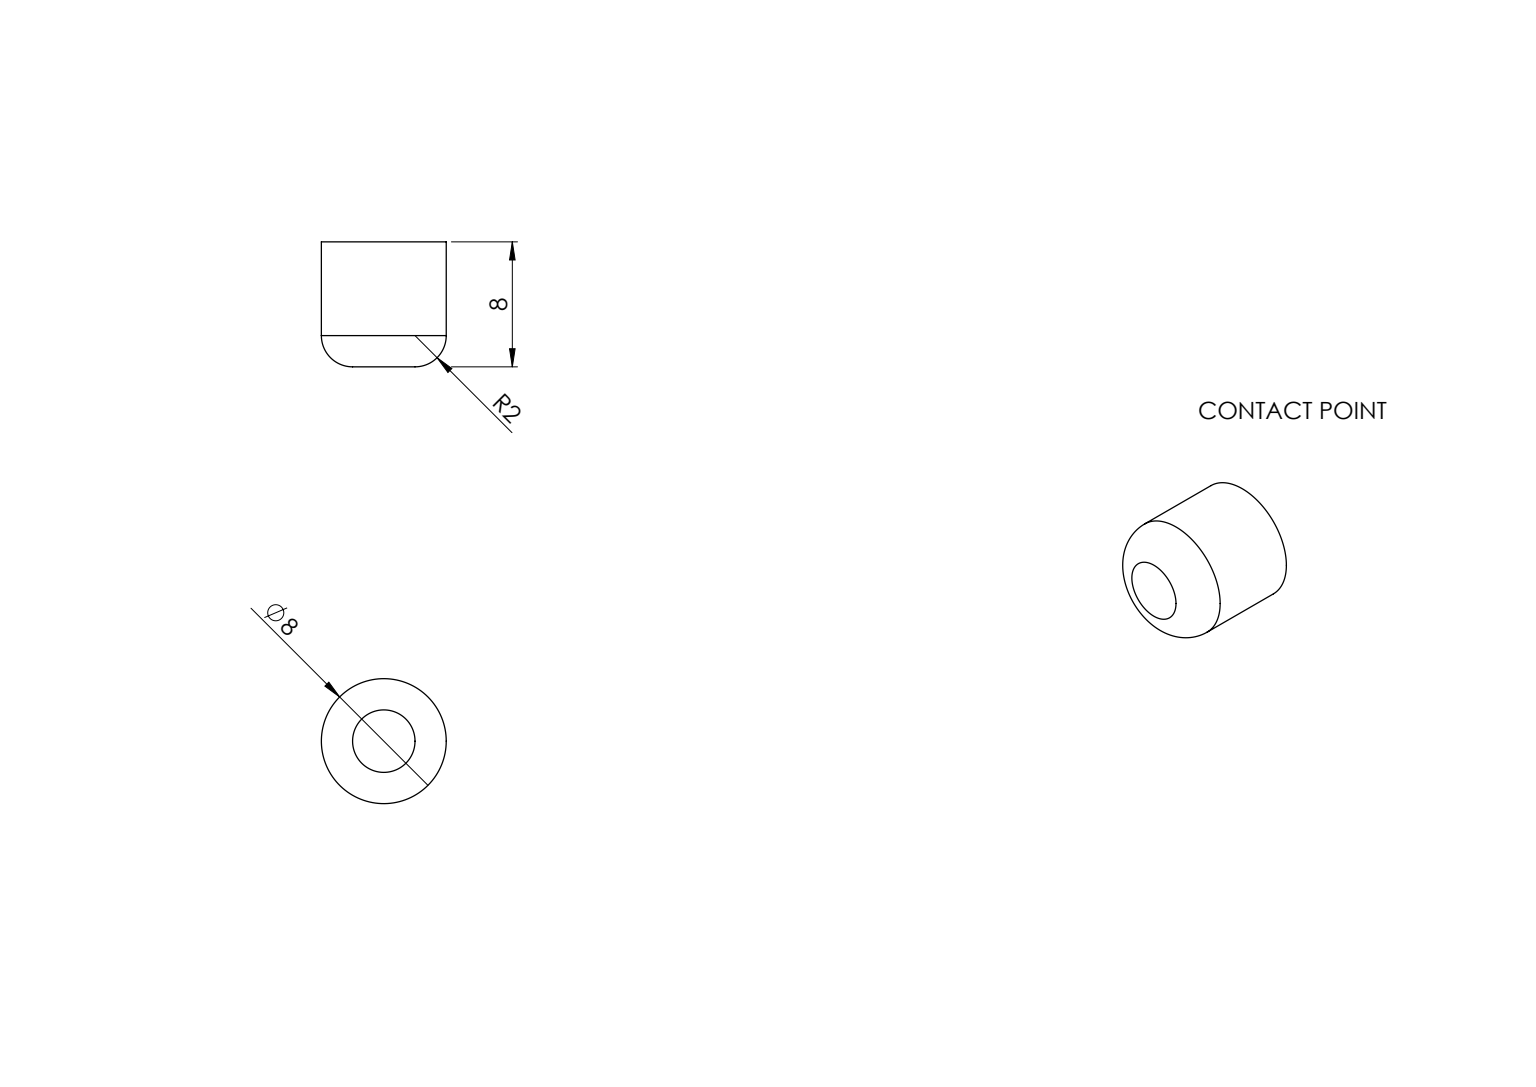
ISO-10303-21;
HEADER;
FILE_DESCRIPTION (('STEP AP214'),
    '1' );
FILE_NAME ('contact point.step',
    '2026-10-26T12:50:16',
    ( '' ),
    ( '' ),
    'SwSTEP 2.0',
    'SolidWorks 2026',
    '' );
FILE_SCHEMA (( 'AUTOMOTIVE_DESIGN' ));
ENDSEC;

DATA;
#29=ORIENTED_EDGE ( 'NONE', *, *, #15667, .T. ) ;
#56=VERTEX_POINT ( 'NONE', #24269 ) ;
#75=TOROIDAL_SURFACE ( 'NONE', #19699, 2.000000000000000000, 2.000000000000000000 ) ;
#102=ADVANCED_FACE ( 'NONE', ( #22181 ), #12564, .T. ) ;
#110=CARTESIAN_POINT ( 'NONE',  ( 1.500000000000001776, -10.49999999999999289, 4.999999999999993783 ) ) ;
#186=ORIENTED_EDGE ( 'NONE', *, *, #6669, .T. ) ;
#197=EDGE_CURVE ( 'NONE', #20602, #23121, #20077, .T. ) ;
#412=ORIENTED_EDGE ( 'NONE', *, *, #15667, .F. ) ;
#459=( GEOMETRIC_REPRESENTATION_CONTEXT ( 3 ) GLOBAL_UNCERTAINTY_ASSIGNED_CONTEXT ( ( #10970 ) ) GLOBAL_UNIT_ASSIGNED_CONTEXT ( ( #23012, #3129, #18575 ) ) REPRESENTATION_CONTEXT ( 'NONE', 'WORKASPACE' ) );
#546=EDGE_CURVE ( 'NONE', #10805, #16184, #12212, .T. ) ;
#620=EDGE_CURVE ( 'NONE', #5209, #6382, #2280, .T. ) ;
#698=ORIENTED_EDGE ( 'NONE', *, *, #8966, .F. ) ;
#734=LINE ( 'NONE', #6878, #984 ) ;
#738=FILL_AREA_STYLE_COLOUR ( '', #17309 ) ;
#806=AXIS2_PLACEMENT_3D ( 'NONE', #20605, #12487, #857 ) ;
#857=DIRECTION ( 'NONE',  ( -1.000000000000000000, 0.000000000000000000, 0.000000000000000000 ) ) ;
#871=SHAPE_REPRESENTATION_RELATIONSHIP ( 'NONE' , 'NONE' ,  #23343, #13495 ) ;
#935=ORIENTED_EDGE ( 'NONE', *, *, #9732, .T. ) ;
#984=VECTOR ( 'NONE', #20472, 1000.000000000000000 ) ;
#1087=VERTEX_POINT ( 'NONE', #6518 ) ;
#1292=UNCERTAINTY_MEASURE_WITH_UNIT (LENGTH_MEASURE( 1.000000000000000082E-05 ), #12896, 'distance_accuracy_value', 'NONE');
#1392=PRODUCT_CONTEXT ( 'NONE', #10427, 'mechanical' ) ;
#1414=ORIENTED_EDGE ( 'NONE', *, *, #7433, .F. ) ;
#1426=MECHANICAL_DESIGN_GEOMETRIC_PRESENTATION_REPRESENTATION('',(#12709),#8113);
#1448=EDGE_LOOP ( 'NONE', ( #25041, #5384, #21791, #23680 ) ) ;
#1535=ORIENTED_EDGE ( 'NONE', *, *, #10759, .F. ) ;
#1546=DIRECTION ( 'NONE',  ( 1.000000000000000000, 0.000000000000000000, 0.000000000000000000 ) ) ;
#1618=EDGE_LOOP ( 'NONE', ( #2456, #10455, #25171, #2324 ) ) ;
#2076=DIRECTION ( 'NONE',  ( 0.000000000000000000, -1.000000000000000000, 0.000000000000000000 ) ) ;
#2122=EDGE_CURVE ( 'NONE', #23121, #13852, #15327, .T. ) ;
#2130=CARTESIAN_POINT ( 'NONE',  ( 4.000000000000003553, -8.999999999999992895, 0.000000000000000000 ) ) ;
#2280=LINE ( 'NONE', #19913, #10677 ) ;
#2308=DIRECTION ( 'NONE',  ( 1.000000000000000000, 0.000000000000000000, 0.000000000000000000 ) ) ;
#2324=ORIENTED_EDGE ( 'NONE', *, *, #620, .F. ) ;
#2456=ORIENTED_EDGE ( 'NONE', *, *, #23666, .F. ) ;
#2478=CARTESIAN_POINT ( 'NONE',  ( 1.500000000000001776, -7.499999999999993783, -6.938893903907228378E-15 ) ) ;
#2560=VECTOR ( 'NONE', #24669, 1000.000000000000000 ) ;
#2573=( NAMED_UNIT ( * ) SI_UNIT ( $, .STERADIAN. ) SOLID_ANGLE_UNIT ( ) );
#2605=EDGE_LOOP ( 'NONE', ( #20644, #21893 ) ) ;
#2676=( GEOMETRIC_REPRESENTATION_CONTEXT ( 3 ) GLOBAL_UNCERTAINTY_ASSIGNED_CONTEXT ( ( #12808 ) ) GLOBAL_UNIT_ASSIGNED_CONTEXT ( ( #3892, #25726, #22442 ) ) REPRESENTATION_CONTEXT ( 'NONE', 'WORKASPACE' ) );
#2786=CARTESIAN_POINT ( 'NONE',  ( 3.469446951953614189E-15, -8.999999999999992895, 6.000000000000000000 ) ) ;
#2807=CARTESIAN_POINT ( 'NONE',  ( 3.469446951953614189E-15, -8.999999999999992895, 0.000000000000000000 ) ) ;
#2920=ORIENTED_EDGE ( 'NONE', *, *, #2122, .F. ) ;
#2933=CIRCLE ( 'NONE', #15893, 4.000000000000000000 ) ;
#2940=EDGE_CURVE ( 'NONE', #20602, #3531, #10020, .T. ) ;
#2999=AXIS2_PLACEMENT_3D ( 'NONE', #9884, #3615, #11585 ) ;
#3099=ADVANCED_FACE ( 'NONE', ( #25038, #19143 ), #9217, .F. ) ;
#3100=DIRECTION ( 'NONE',  ( 0.000000000000000000, 0.000000000000000000, 1.000000000000000000 ) ) ;
#3129=( NAMED_UNIT ( * ) PLANE_ANGLE_UNIT ( ) SI_UNIT ( $, .RADIAN. ) );
#3313=EDGE_LOOP ( 'NONE', ( #412, #21152, #3951, #4447 ) ) ;
#3349=CARTESIAN_POINT ( 'NONE',  ( 1.500000000000001776, -7.499999999999993783, 4.999999999999993783 ) ) ;
#3531=VERTEX_POINT ( 'NONE', #23628 ) ;
#3615=DIRECTION ( 'NONE',  ( -0.000000000000000000, -0.000000000000000000, -1.000000000000000000 ) ) ;
#3722=PRODUCT_DEFINITION ( 'UNKNOWN', '', #21072, #20916 ) ;
#3755=DIRECTION ( 'NONE',  ( 0.000000000000000000, 1.000000000000000000, 0.000000000000000000 ) ) ;
#3773=EDGE_LOOP ( 'NONE', ( #1414, #13122, #6814, #9882 ) ) ;
#3789=LINE ( 'NONE', #9159, #13919 ) ;
#3892=( LENGTH_UNIT ( ) NAMED_UNIT ( * ) SI_UNIT ( .MILLI., .METRE. ) );
#3951=ORIENTED_EDGE ( 'NONE', *, *, #2122, .T. ) ;
#4029=PLANE ( 'NONE',  #25126 ) ;
#4157=DIRECTION ( 'NONE',  ( -1.000000000000000000, 0.000000000000000000, 0.000000000000000000 ) ) ;
#4231=CIRCLE ( 'NONE', #6325, 2.000000000000000000 ) ;
#4279=LINE ( 'NONE', #110, #15026 ) ;
#4314=DIRECTION ( 'NONE',  ( 1.000000000000000000, -0.000000000000000000, -0.000000000000000000 ) ) ;
#4383=EDGE_LOOP ( 'NONE', ( #19500, #13715, #698, #5012 ) ) ;
#4403=CYLINDRICAL_SURFACE ( 'NONE', #8424, 4.000000000000000000 ) ;
#4447=ORIENTED_EDGE ( 'NONE', *, *, #10150, .T. ) ;
#4601=DIRECTION ( 'NONE',  ( 0.000000000000000000, 1.000000000000000000, 0.000000000000000000 ) ) ;
#4751=CARTESIAN_POINT ( 'NONE',  ( 1.500000000000001776, -10.49999999999999289, -6.938893903907228378E-15 ) ) ;
#4765=FACE_OUTER_BOUND ( 'NONE', #4383, .T. ) ;
#4835=FACE_OUTER_BOUND ( 'NONE', #1448, .T. ) ;
#4917=FACE_OUTER_BOUND ( 'NONE', #9792, .T. ) ;
#5012=ORIENTED_EDGE ( 'NONE', *, *, #2940, .F. ) ;
#5149=DIRECTION ( 'NONE',  ( 0.000000000000000000, 0.000000000000000000, 1.000000000000000000 ) ) ;
#5173=DIRECTION ( 'NONE',  ( 0.000000000000000000, 0.000000000000000000, 1.000000000000000000 ) ) ;
#5209=VERTEX_POINT ( 'NONE', #6579 ) ;
#5233=EDGE_CURVE ( 'NONE', #5209, #1087, #7239, .T. ) ;
#5384=ORIENTED_EDGE ( 'NONE', *, *, #5233, .F. ) ;
#5442=MECHANICAL_DESIGN_GEOMETRIC_PRESENTATION_REPRESENTATION('',(#23407),#459);
#5468=DIRECTION ( 'NONE',  ( 0.000000000000000000, 0.000000000000000000, 1.000000000000000000 ) ) ;
#5632=DIRECTION ( 'NONE',  ( 0.000000000000000000, 0.000000000000000000, 1.000000000000000000 ) ) ;
#5687=EDGE_CURVE ( 'NONE', #7768, #17145, #734, .T. ) ;
#5822=FACE_OUTER_BOUND ( 'NONE', #12954, .T. ) ;
#5941=CARTESIAN_POINT ( 'NONE',  ( 1.500000000000001776, -7.499999999999993783, 4.999999999999993783 ) ) ;
#5971=DIRECTION ( 'NONE',  ( -0.000000000000000000, -0.000000000000000000, -1.000000000000000000 ) ) ;
#5983=PLANE ( 'NONE',  #22192 ) ;
#6120=CARTESIAN_POINT ( 'NONE',  ( 1.500000000000001776, -10.49999999999999289, 4.999999999999993783 ) ) ;
#6325=AXIS2_PLACEMENT_3D ( 'NONE', #13043, #3100, #11959 ) ;
#6372=CARTESIAN_POINT ( 'NONE',  ( 3.469446951953614189E-15, -8.999999999999992895, 8.000000000000000000 ) ) ;
#6382=VERTEX_POINT ( 'NONE', #15341 ) ;
#6402=CARTESIAN_POINT ( 'NONE',  ( -3.999999999999996447, -8.999999999999992895, 6.000000000000000000 ) ) ;
#6518=CARTESIAN_POINT ( 'NONE',  ( -1.499999999999998224, -10.49999999999999289, -6.938893903907228378E-15 ) ) ;
#6579=CARTESIAN_POINT ( 'NONE',  ( -1.499999999999998224, -10.49999999999999289, 4.999999999999993783 ) ) ;
#6629=CARTESIAN_POINT ( 'NONE',  ( 3.469446951953614189E-15, -8.999999999999992895, 8.000000000000000000 ) ) ;
#6669=EDGE_CURVE ( 'NONE', #23121, #20602, #23055, .T. ) ;
#6814=ORIENTED_EDGE ( 'NONE', *, *, #12872, .T. ) ;
#6878=CARTESIAN_POINT ( 'NONE',  ( 1.500000000000001776, -7.499999999999993783, -6.938893903907228378E-15 ) ) ;
#6882=SURFACE_STYLE_USAGE ( .BOTH. , #8708 ) ;
#6884=CARTESIAN_POINT ( 'NONE',  ( -1.499999999999998224, -10.49999999999999289, 4.999999999999993783 ) ) ;
#6906=ADVANCED_FACE ( 'NONE', ( #4765 ), #75, .T. ) ;
#7004=( NAMED_UNIT ( * ) PLANE_ANGLE_UNIT ( ) SI_UNIT ( $, .RADIAN. ) );
#7052=AXIS2_PLACEMENT_3D ( 'NONE', #21524, #21788, #15381 ) ;
#7095=ORIENTED_EDGE ( 'NONE', *, *, #23089, .T. ) ;
#7203=ORIENTED_EDGE ( 'NONE', *, *, #7433, .T. ) ;
#7239=LINE ( 'NONE', #15088, #20162 ) ;
#7312=PLANE ( 'NONE',  #22650 ) ;
#7346=DIRECTION ( 'NONE',  ( -0.000000000000000000, -0.000000000000000000, -1.000000000000000000 ) ) ;
#7356=VECTOR ( 'NONE', #14320, 1000.000000000000000 ) ;
#7433=EDGE_CURVE ( 'NONE', #19275, #7768, #10613, .T. ) ;
#7597=CARTESIAN_POINT ( 'NONE',  ( 3.469446951953614189E-15, -8.999999999999992895, 0.000000000000000000 ) ) ;
#7722=DIRECTION ( 'NONE',  ( 1.000000000000000000, 0.000000000000000000, 0.000000000000000000 ) ) ;
#7768=VERTEX_POINT ( 'NONE', #2478 ) ;
#7873=FACE_OUTER_BOUND ( 'NONE', #15677, .T. ) ;
#7961=CARTESIAN_POINT ( 'NONE',  ( 2.000000000000003553, -8.999999999999992895, 6.000000000000000000 ) ) ;
#7967=PRODUCT ( 'contact point', 'contact point', '', ( #1392 ) ) ;
#7974=ADVANCED_FACE ( 'NONE', ( #4835 ), #7312, .T. ) ;
#8082=CARTESIAN_POINT ( 'NONE',  ( 0.000000000000000000, 0.000000000000000000, 4.999999999999993783 ) ) ;
#8113=( GEOMETRIC_REPRESENTATION_CONTEXT ( 3 ) GLOBAL_UNCERTAINTY_ASSIGNED_CONTEXT ( ( #1292 ) ) GLOBAL_UNIT_ASSIGNED_CONTEXT ( ( #12896, #7004, #2573 ) ) REPRESENTATION_CONTEXT ( 'NONE', 'WORKASPACE' ) );
#8210=ORIENTED_EDGE ( 'NONE', *, *, #546, .T. ) ;
#8424=AXIS2_PLACEMENT_3D ( 'NONE', #6372, #16698, #16455 ) ;
#8426=EDGE_LOOP ( 'NONE', ( #20466, #13566, #8210, #10955 ) ) ;
#8482=FACE_OUTER_BOUND ( 'NONE', #3773, .T. ) ;
#8651=CARTESIAN_POINT ( 'NONE',  ( -1.499999999999998224, -10.49999999999999289, -6.938893903907228378E-15 ) ) ;
#8708=SURFACE_SIDE_STYLE ('',( #10540 ) ) ;
#8739=CIRCLE ( 'NONE', #806, 2.000000000000000000 ) ;
#8828=AXIS2_PLACEMENT_3D ( 'NONE', #6629, #22855, #10806 ) ;
#8935=LINE ( 'NONE', #20816, #17185 ) ;
#8966=EDGE_CURVE ( 'NONE', #3531, #56, #11404, .T. ) ;
#8968=DIRECTION ( 'NONE',  ( 1.000000000000000000, 0.000000000000000000, -0.000000000000000000 ) ) ;
#9159=CARTESIAN_POINT ( 'NONE',  ( 1.500000000000001776, -10.49999999999999289, 4.999999999999993783 ) ) ;
#9186=CARTESIAN_POINT ( 'NONE',  ( 4.000000000000003553, -8.999999999999992895, 6.000000000000000000 ) ) ;
#9217=PLANE ( 'NONE',  #23808 ) ;
#9314=LINE ( 'NONE', #17299, #15374 ) ;
#9588=VERTEX_POINT ( 'NONE', #2130 ) ;
#9625=LINE ( 'NONE', #3349, #14167 ) ;
#9722=ADVANCED_FACE ( 'NONE', ( #7873 ), #14032, .T. ) ;
#9732=EDGE_CURVE ( 'NONE', #17145, #1087, #14676, .T. ) ;
#9792=EDGE_LOOP ( 'NONE', ( #186, #29, #20419, #2920 ) ) ;
#9811=LINE ( 'NONE', #14262, #23836 ) ;
#9882=ORIENTED_EDGE ( 'NONE', *, *, #16665, .T. ) ;
#9884=CARTESIAN_POINT ( 'NONE',  ( 3.469446951953614189E-15, -8.999999999999992895, 6.000000000000000000 ) ) ;
#10020=CIRCLE ( 'NONE', #13789, 2.000000000000000000 ) ;
#10144=ORIENTED_EDGE ( 'NONE', *, *, #2940, .T. ) ;
#10150=EDGE_CURVE ( 'NONE', #13852, #9588, #24700, .T. ) ;
#10158=DIRECTION ( 'NONE',  ( 0.000000000000000000, -0.000000000000000000, 1.000000000000000000 ) ) ;
#10316=ADVANCED_FACE ( 'NONE', ( #16178 ), #5983, .F. ) ;
#10427=APPLICATION_CONTEXT ( 'automotive_design' ) ;
#10438=ADVANCED_FACE ( 'NONE', ( #4917 ), #4403, .T. ) ;
#10455=ORIENTED_EDGE ( 'NONE', *, *, #546, .F. ) ;
#10457=CARTESIAN_POINT ( 'NONE',  ( 1.500000000000001776, -7.499999999999993783, 4.999999999999993783 ) ) ;
#10459=AXIS2_PLACEMENT_3D ( 'NONE', #22381, #24217, #22263 ) ;
#10499=VECTOR ( 'NONE', #4601, 1000.000000000000000 ) ;
#10540=SURFACE_STYLE_FILL_AREA ( #24926 ) ;
#10613=LINE ( 'NONE', #4751, #10499 ) ;
#10677=VECTOR ( 'NONE', #18355, 1000.000000000000000 ) ;
#10759=EDGE_CURVE ( 'NONE', #16184, #17145, #8935, .T. ) ;
#10805=VERTEX_POINT ( 'NONE', #23391 ) ;
#10806=DIRECTION ( 'NONE',  ( -1.000000000000000000, 0.000000000000000000, 0.000000000000000000 ) ) ;
#10955=ORIENTED_EDGE ( 'NONE', *, *, #10759, .T. ) ;
#10970=UNCERTAINTY_MEASURE_WITH_UNIT (LENGTH_MEASURE( 1.000000000000000082E-05 ), #23012, 'distance_accuracy_value', 'NONE');
#11129=DIRECTION ( 'NONE',  ( -0.000000000000000000, -0.000000000000000000, -1.000000000000000000 ) ) ;
#11241=DIRECTION ( 'NONE',  ( -0.000000000000000000, -0.000000000000000000, -1.000000000000000000 ) ) ;
#11349=EDGE_CURVE ( 'NONE', #56, #3531, #4231, .T. ) ;
#11404=CIRCLE ( 'NONE', #14751, 2.000000000000000000 ) ;
#11585=DIRECTION ( 'NONE',  ( 1.000000000000000000, 0.000000000000000000, 0.000000000000000000 ) ) ;
#11691=ADVANCED_FACE ( 'NONE', ( #8482 ), #4029, .T. ) ;
#11748=CARTESIAN_POINT ( 'NONE',  ( -1.499999999999998224, -7.499999999999992895, 4.999999999999993783 ) ) ;
#11861=ADVANCED_FACE ( 'NONE', ( #20496 ), #24429, .T. ) ;
#11959=DIRECTION ( 'NONE',  ( 1.000000000000000000, 0.000000000000000000, 0.000000000000000000 ) ) ;
#12212=LINE ( 'NONE', #5941, #7356 ) ;
#12302=PLANE ( 'NONE',  #22941 ) ;
#12487=DIRECTION ( 'NONE',  ( 1.224646799147353207E-16, 1.000000000000000000, -0.000000000000000000 ) ) ;
#12556=DIRECTION ( 'NONE',  ( 1.000000000000000000, -2.891205793294678326E-16, 0.000000000000000000 ) ) ;
#12564=TOROIDAL_SURFACE ( 'NONE', #14664, 2.000000000000000000, 2.000000000000000000 ) ;
#12578=AXIS2_PLACEMENT_3D ( 'NONE', #13195, #5468, #1546 ) ;
#12618=APPLICATION_CONTEXT ( 'automotive_design' ) ;
#12709=STYLED_ITEM ( 'NONE', ( #22967 ), #13495 ) ;
#12808=UNCERTAINTY_MEASURE_WITH_UNIT (LENGTH_MEASURE( 1.000000000000000082E-05 ), #3892, 'distance_accuracy_value', 'NONE');
#12872=EDGE_CURVE ( 'NONE', #6382, #10805, #4279, .T. ) ;
#12896=( LENGTH_UNIT ( ) NAMED_UNIT ( * ) SI_UNIT ( .MILLI., .METRE. ) );
#12954=EDGE_LOOP ( 'NONE', ( #22366, #18978 ) ) ;
#13043=CARTESIAN_POINT ( 'NONE',  ( 3.469446951953614189E-15, -8.999999999999992895, 8.000000000000000000 ) ) ;
#13122=ORIENTED_EDGE ( 'NONE', *, *, #25683, .F. ) ;
#13195=CARTESIAN_POINT ( 'NONE',  ( 3.469446951953614189E-15, -8.999999999999992895, 0.000000000000000000 ) ) ;
#13223=DIRECTION ( 'NONE',  ( 1.000000000000000000, 0.000000000000000000, 0.000000000000000000 ) ) ;
#13353=CARTESIAN_POINT ( 'NONE',  ( 0.000000000000000000, 0.000000000000000000, 0.000000000000000000 ) ) ;
#13495=ADVANCED_BREP_SHAPE_REPRESENTATION ( '', ( #14010, #21036 ), #2676 ) ;
#13558=PLANE ( 'NONE',  #7052 ) ;
#13566=ORIENTED_EDGE ( 'NONE', *, *, #16665, .F. ) ;
#13715=ORIENTED_EDGE ( 'NONE', *, *, #21059, .T. ) ;
#13789=AXIS2_PLACEMENT_3D ( 'NONE', #7961, #2076, #15947 ) ;
#13852=VERTEX_POINT ( 'NONE', #24451 ) ;
#13919=VECTOR ( 'NONE', #11241, 1000.000000000000000 ) ;
#13954=DIRECTION ( 'NONE',  ( 1.000000000000000000, 0.000000000000000000, 0.000000000000000000 ) ) ;
#14010=MANIFOLD_SOLID_BREP ( 'Cavity1', #23820 ) ;
#14032=PLANE ( 'NONE',  #10459 ) ;
#14167=VECTOR ( 'NONE', #25207, 1000.000000000000000 ) ;
#14253=VECTOR ( 'NONE', #22124, 1000.000000000000000 ) ;
#14262=CARTESIAN_POINT ( 'NONE',  ( 1.500000000000001776, -10.49999999999999289, -6.938893903907228378E-15 ) ) ;
#14320=DIRECTION ( 'NONE',  ( -1.000000000000000000, 2.891205793294678326E-16, 0.000000000000000000 ) ) ;
#14664=AXIS2_PLACEMENT_3D ( 'NONE', #18385, #16049, #2308 ) ;
#14676=LINE ( 'NONE', #8651, #14253 ) ;
#14751=AXIS2_PLACEMENT_3D ( 'NONE', #21441, #17770, #25739 ) ;
#14906=DIRECTION ( 'NONE',  ( 0.000000000000000000, 0.000000000000000000, 1.000000000000000000 ) ) ;
#15026=VECTOR ( 'NONE', #3755, 1000.000000000000000 ) ;
#15088=CARTESIAN_POINT ( 'NONE',  ( -1.499999999999998224, -10.49999999999999289, 4.999999999999993783 ) ) ;
#15133=SHAPE_DEFINITION_REPRESENTATION ( #17993, #23343 ) ;
#15173=DIRECTION ( 'NONE',  ( 0.000000000000000000, 1.000000000000000000, -0.000000000000000000 ) ) ;
#15289=CARTESIAN_POINT ( 'NONE',  ( 1.500000000000001776, -10.49999999999999289, 4.999999999999993783 ) ) ;
#15327=LINE ( 'NONE', #25141, #18361 ) ;
#15341=CARTESIAN_POINT ( 'NONE',  ( 1.500000000000001776, -10.49999999999999289, 4.999999999999993783 ) ) ;
#15374=VECTOR ( 'NONE', #7346, 1000.000000000000000 ) ;
#15381=DIRECTION ( 'NONE',  ( 1.000000000000000000, 0.000000000000000000, -0.000000000000000000 ) ) ;
#15433=ORIENTED_EDGE ( 'NONE', *, *, #11349, .F. ) ;
#15667=EDGE_CURVE ( 'NONE', #20602, #9588, #9314, .T. ) ;
#15677=EDGE_LOOP ( 'NONE', ( #22101, #1535, #23739, #18528 ) ) ;
#15703=DIRECTION ( 'NONE',  ( 0.000000000000000000, 0.000000000000000000, 1.000000000000000000 ) ) ;
#15893=AXIS2_PLACEMENT_3D ( 'NONE', #7597, #5632, #7722 ) ;
#15945=DIRECTION ( 'NONE',  ( 0.000000000000000000, 0.000000000000000000, 1.000000000000000000 ) ) ;
#15947=DIRECTION ( 'NONE',  ( 0.000000000000000000, 0.000000000000000000, -1.000000000000000000 ) ) ;
#16049=DIRECTION ( 'NONE',  ( 0.000000000000000000, 0.000000000000000000, 1.000000000000000000 ) ) ;
#16178=FACE_OUTER_BOUND ( 'NONE', #1618, .T. ) ;
#16184=VERTEX_POINT ( 'NONE', #11748 ) ;
#16455=DIRECTION ( 'NONE',  ( -1.000000000000000000, 0.000000000000000000, 0.000000000000000000 ) ) ;
#16665=EDGE_CURVE ( 'NONE', #10805, #7768, #9625, .T. ) ;
#16698=DIRECTION ( 'NONE',  ( -0.000000000000000000, -0.000000000000000000, -1.000000000000000000 ) ) ;
#16726=ADVANCED_FACE ( 'NONE', ( #5822 ), #13558, .T. ) ;
#16793=EDGE_LOOP ( 'NONE', ( #935, #7095, #7203, #24654 ) ) ;
#16794=DIRECTION ( 'NONE',  ( 1.000000000000000000, 0.000000000000000000, 0.000000000000000000 ) ) ;
#17046=ADVANCED_FACE ( 'NONE', ( #24198 ), #12302, .T. ) ;
#17145=VERTEX_POINT ( 'NONE', #22104 ) ;
#17185=VECTOR ( 'NONE', #11129, 1000.000000000000000 ) ;
#17299=CARTESIAN_POINT ( 'NONE',  ( 4.000000000000003553, -8.999999999999992895, 8.000000000000000000 ) ) ;
#17309=COLOUR_RGB ( '',0.8941176470588234615, 0.8941176470588234615, 0.8941176470588234615 ) ;
#17664=DIRECTION ( 'NONE',  ( -0.000000000000000000, -0.000000000000000000, -1.000000000000000000 ) ) ;
#17770=DIRECTION ( 'NONE',  ( 0.000000000000000000, 0.000000000000000000, 1.000000000000000000 ) ) ;
#17883=DIRECTION ( 'NONE',  ( 1.000000000000000000, 0.000000000000000000, -0.000000000000000000 ) ) ;
#17993=PRODUCT_DEFINITION_SHAPE ( 'NONE', 'NONE',  #3722 ) ;
#18355=DIRECTION ( 'NONE',  ( 1.000000000000000000, -0.000000000000000000, -0.000000000000000000 ) ) ;
#18361=VECTOR ( 'NONE', #23297, 1000.000000000000000 ) ;
#18385=CARTESIAN_POINT ( 'NONE',  ( 3.469446951953614189E-15, -8.999999999999992895, 6.000000000000000000 ) ) ;
#18528=ORIENTED_EDGE ( 'NONE', *, *, #5233, .T. ) ;
#18575=( NAMED_UNIT ( * ) SI_UNIT ( $, .STERADIAN. ) SOLID_ANGLE_UNIT ( ) );
#18978=ORIENTED_EDGE ( 'NONE', *, *, #11349, .T. ) ;
#19143=FACE_BOUND ( 'NONE', #16793, .T. ) ;
#19275=VERTEX_POINT ( 'NONE', #20532 ) ;
#19437=ORIENTED_EDGE ( 'NONE', *, *, #21059, .F. ) ;
#19500=ORIENTED_EDGE ( 'NONE', *, *, #6669, .F. ) ;
#19699=AXIS2_PLACEMENT_3D ( 'NONE', #2786, #5149, #16794 ) ;
#19913=CARTESIAN_POINT ( 'NONE',  ( 1.500000000000001776, -10.49999999999999289, 4.999999999999993783 ) ) ;
#20077=CIRCLE ( 'NONE', #22591, 4.000000000000000000 ) ;
#20162=VECTOR ( 'NONE', #17664, 1000.000000000000000 ) ;
#20268=DIRECTION ( 'NONE',  ( -2.891205793294678326E-16, -1.000000000000000000, 0.000000000000000000 ) ) ;
#20419=ORIENTED_EDGE ( 'NONE', *, *, #22936, .T. ) ;
#20466=ORIENTED_EDGE ( 'NONE', *, *, #5687, .F. ) ;
#20472=DIRECTION ( 'NONE',  ( -1.000000000000000000, 2.891205793294678326E-16, 0.000000000000000000 ) ) ;
#20496=FACE_OUTER_BOUND ( 'NONE', #3313, .T. ) ;
#20532=CARTESIAN_POINT ( 'NONE',  ( 1.500000000000001776, -10.49999999999999289, -6.938893903907228378E-15 ) ) ;
#20602=VERTEX_POINT ( 'NONE', #9186 ) ;
#20605=CARTESIAN_POINT ( 'NONE',  ( -1.999999999999996669, -8.999999999999992895, 6.000000000000000000 ) ) ;
#20644=ORIENTED_EDGE ( 'NONE', *, *, #10150, .F. ) ;
#20816=CARTESIAN_POINT ( 'NONE',  ( -1.499999999999998224, -7.499999999999992895, 4.999999999999993783 ) ) ;
#20916=PRODUCT_DEFINITION_CONTEXT ( 'detailed design', #12618, 'design' ) ;
#21036=AXIS2_PLACEMENT_3D ( 'NONE', #13353, #15703, #13223 ) ;
#21059=EDGE_CURVE ( 'NONE', #23121, #56, #8739, .T. ) ;
#21072=PRODUCT_DEFINITION_FORMATION_WITH_SPECIFIED_SOURCE ( 'ANY', '', #7967, .NOT_KNOWN. ) ;
#21152=ORIENTED_EDGE ( 'NONE', *, *, #197, .T. ) ;
#21441=CARTESIAN_POINT ( 'NONE',  ( 3.469446951953614189E-15, -8.999999999999992895, 8.000000000000000000 ) ) ;
#21524=CARTESIAN_POINT ( 'NONE',  ( 3.469446951953614189E-15, -8.999999999999992895, 8.000000000000000000 ) ) ;
#21788=DIRECTION ( 'NONE',  ( 0.000000000000000000, 0.000000000000000000, 1.000000000000000000 ) ) ;
#21791=ORIENTED_EDGE ( 'NONE', *, *, #620, .T. ) ;
#21893=ORIENTED_EDGE ( 'NONE', *, *, #22936, .F. ) ;
#22101=ORIENTED_EDGE ( 'NONE', *, *, #9732, .F. ) ;
#22104=CARTESIAN_POINT ( 'NONE',  ( -1.499999999999998224, -7.499999999999992006, 0.000000000000000000 ) ) ;
#22124=DIRECTION ( 'NONE',  ( -0.000000000000000000, -1.000000000000000000, -0.000000000000000000 ) ) ;
#22181=FACE_OUTER_BOUND ( 'NONE', #24405, .T. ) ;
#22192=AXIS2_PLACEMENT_3D ( 'NONE', #8082, #10158, #17883 ) ;
#22263=DIRECTION ( 'NONE',  ( 0.000000000000000000, 0.000000000000000000, -1.000000000000000000 ) ) ;
#22366=ORIENTED_EDGE ( 'NONE', *, *, #8966, .T. ) ;
#22381=CARTESIAN_POINT ( 'NONE',  ( -1.499999999999998224, -10.49999999999999289, 4.999999999999993783 ) ) ;
#22442=( NAMED_UNIT ( * ) SI_UNIT ( $, .STERADIAN. ) SOLID_ANGLE_UNIT ( ) );
#22591=AXIS2_PLACEMENT_3D ( 'NONE', #23889, #5971, #13954 ) ;
#22650=AXIS2_PLACEMENT_3D ( 'NONE', #15289, #15173, #14906 ) ;
#22855=DIRECTION ( 'NONE',  ( -0.000000000000000000, -0.000000000000000000, -1.000000000000000000 ) ) ;
#22936=EDGE_CURVE ( 'NONE', #9588, #13852, #2933, .T. ) ;
#22941=AXIS2_PLACEMENT_3D ( 'NONE', #10457, #20268, #12556 ) ;
#22967=PRESENTATION_STYLE_ASSIGNMENT (( #6882 ) ) ;
#23012=( LENGTH_UNIT ( ) NAMED_UNIT ( * ) SI_UNIT ( .MILLI., .METRE. ) );
#23055=CIRCLE ( 'NONE', #2999, 4.000000000000000000 ) ;
#23089=EDGE_CURVE ( 'NONE', #1087, #19275, #9811, .T. ) ;
#23121=VERTEX_POINT ( 'NONE', #6402 ) ;
#23297=DIRECTION ( 'NONE',  ( -0.000000000000000000, -0.000000000000000000, -1.000000000000000000 ) ) ;
#23343=SHAPE_REPRESENTATION ( 'contact point', ( #21036 ), #2676 ) ;
#23391=CARTESIAN_POINT ( 'NONE',  ( 1.500000000000001776, -7.499999999999993783, 4.999999999999993783 ) ) ;
#23407=STYLED_ITEM('',(#25907),#14010);
#23628=CARTESIAN_POINT ( 'NONE',  ( 2.000000000000003553, -8.999999999999992895, 8.000000000000000000 ) ) ;
#23666=EDGE_CURVE ( 'NONE', #16184, #5209, #24286, .T. ) ;
#23680=ORIENTED_EDGE ( 'NONE', *, *, #25683, .T. ) ;
#23739=ORIENTED_EDGE ( 'NONE', *, *, #23666, .T. ) ;
#23808=AXIS2_PLACEMENT_3D ( 'NONE', #2807, #5173, #8968 ) ;
#23820=CLOSED_SHELL ( 'NONE', ( #6906, #10438, #3099, #11861, #16726, #102, #9722, #7974, #11691, #17046, #10316 ) ) ;
#23836=VECTOR ( 'NONE', #4314, 1000.000000000000000 ) ;
#23889=CARTESIAN_POINT ( 'NONE',  ( 3.469446951953614189E-15, -8.999999999999992895, 6.000000000000000000 ) ) ;
#24198=FACE_OUTER_BOUND ( 'NONE', #8426, .T. ) ;
#24217=DIRECTION ( 'NONE',  ( 1.000000000000000000, 0.000000000000000000, 0.000000000000000000 ) ) ;
#24269=CARTESIAN_POINT ( 'NONE',  ( -1.999999999999996669, -8.999999999999992895, 8.000000000000000000 ) ) ;
#24286=LINE ( 'NONE', #6884, #2560 ) ;
#24405=EDGE_LOOP ( 'NONE', ( #19437, #24468, #10144, #15433 ) ) ;
#24429=CYLINDRICAL_SURFACE ( 'NONE', #8828, 4.000000000000000000 ) ;
#24451=CARTESIAN_POINT ( 'NONE',  ( -3.999999999999996447, -8.999999999999992895, 0.000000000000000000 ) ) ;
#24468=ORIENTED_EDGE ( 'NONE', *, *, #197, .F. ) ;
#24654=ORIENTED_EDGE ( 'NONE', *, *, #5687, .T. ) ;
#24669=DIRECTION ( 'NONE',  ( -0.000000000000000000, -1.000000000000000000, -0.000000000000000000 ) ) ;
#24700=CIRCLE ( 'NONE', #12578, 4.000000000000000000 ) ;
#24926=FILL_AREA_STYLE ('',( #738 ) ) ;
#25038=FACE_OUTER_BOUND ( 'NONE', #2605, .T. ) ;
#25041=ORIENTED_EDGE ( 'NONE', *, *, #23089, .F. ) ;
#25126=AXIS2_PLACEMENT_3D ( 'NONE', #6120, #4157, #15945 ) ;
#25141=CARTESIAN_POINT ( 'NONE',  ( -3.999999999999996447, -8.999999999999992895, 8.000000000000000000 ) ) ;
#25171=ORIENTED_EDGE ( 'NONE', *, *, #12872, .F. ) ;
#25207=DIRECTION ( 'NONE',  ( -0.000000000000000000, -0.000000000000000000, -1.000000000000000000 ) ) ;
#25683=EDGE_CURVE ( 'NONE', #6382, #19275, #3789, .T. ) ;
#25726=( NAMED_UNIT ( * ) PLANE_ANGLE_UNIT ( ) SI_UNIT ( $, .RADIAN. ) );
#25739=DIRECTION ( 'NONE',  ( 1.000000000000000000, 0.000000000000000000, 0.000000000000000000 ) ) ;
#25901=COLOUR_RGB('Sky Blue',0.24,0.69,0.87);
#25902=FILL_AREA_STYLE_COLOUR('',#25901);
#25903=FILL_AREA_STYLE('',(#25902));
#25904=SURFACE_STYLE_FILL_AREA(#25903);
#25905=SURFACE_SIDE_STYLE('',(#25904));
#25906=SURFACE_STYLE_USAGE(.BOTH.,#25905);
#25907=PRESENTATION_STYLE_ASSIGNMENT((#25906));
ENDSEC;
END-ISO-10303-21;
